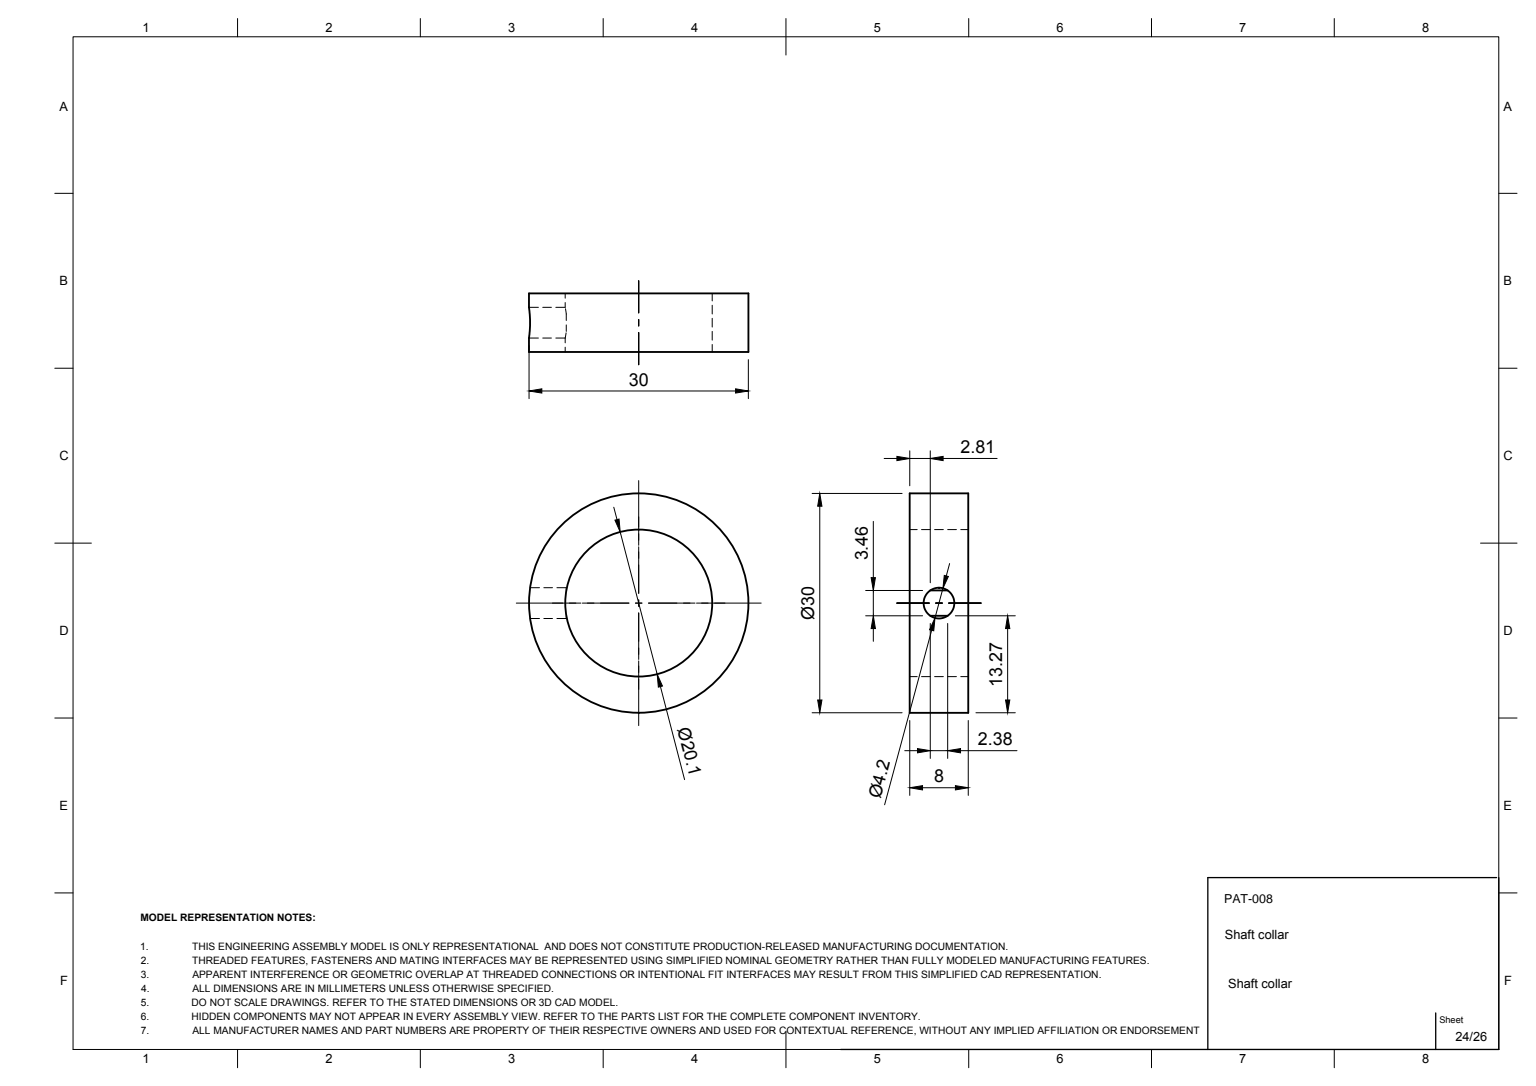
ISO-10303-21;
HEADER;
/* Generated by software containing ST-Developer
 * from STEP Tools, Inc. (www.steptools.com) 
 */

FILE_DESCRIPTION(
/* description */ ('Bearing housing with oil seal and end cap'),
/* implementation_level */ '2;1');

FILE_NAME(
/* name */ 'Shaft collar.step',
/* time_stamp */ '2026-10-28T03:23:10-07:00',
/* author */ (''),
/* organization */ (''),
/* preprocessor_version */ 'ST-DEVELOPER v20.2',
/* originating_system */ 'Autodesk Translation Framework v15.17.0.0',
/* authorisation */ '');

FILE_SCHEMA (('AUTOMOTIVE_DESIGN { 1 0 10303 214 3 1 1 }'));
ENDSEC;

DATA;
#10=MECHANICAL_DESIGN_GEOMETRIC_PRESENTATION_REPRESENTATION('',(#284),#7871);
#177=B_SPLINE_CURVE_WITH_KNOTS('',3,(#7483,#7484,#7485,#7486,#7487,#7488,
#7489,#7490,#7491,#7492,#7493,#7494,#7495,#7496),.UNSPECIFIED.,.F.,.F.,
(4,2,2,2,2,2,4),(0.756005737987012,0.793568827564648,0.872922520054202,
0.952276212543757,1.03162990503331,1.11098359752287,1.1485466871005),
 .UNSPECIFIED.);
#178=B_SPLINE_CURVE_WITH_KNOTS('',3,(#7502,#7503,#7504,#7505,#7506,#7507,
#7508,#7509,#7510,#7511,#7512,#7513,#7514,#7515,#7516,#7517,#7518,#7519),
 .UNSPECIFIED.,.F.,.F.,(4,2,2,2,2,2,2,2,4),(0.,0.0792165807733632,0.158433161546726,
0.237648697074571,0.316864232602415,0.396079768130259,0.475295303658103,
0.554511884431466,0.63372846520483),.UNSPECIFIED.);
#179=B_SPLINE_CURVE_WITH_KNOTS('',3,(#7520,#7521,#7522,#7523,#7524,#7525,
#7526,#7527,#7528,#7529,#7530,#7531,#7532,#7533,#7534,#7535,#7536,#7537),
 .UNSPECIFIED.,.F.,.F.,(4,2,2,2,2,2,2,2,4),(0.63372846520483,0.712945045978192,
0.792161626751555,0.8713771622794,0.950592697807244,1.02980823333509,1.10902376886293,
1.1882403496363,1.26745693040966),.UNSPECIFIED.);
#180=B_SPLINE_CURVE_WITH_KNOTS('',3,(#7540,#7541,#7542,#7543,#7544,#7545,
#7546,#7547,#7548,#7549,#7550,#7551,#7552,#7553),.UNSPECIFIED.,.F.,.F.,
(4,2,2,2,2,2,4),(0.121154929624506,0.158718019202143,0.238071711691698,
0.317425404181252,0.396779096670807,0.476132789160362,0.513695878737999),
 .UNSPECIFIED.);
#234=SHAPE_REPRESENTATION_RELATIONSHIP('SRR','None',#7983,#255);
#255=ADVANCED_BREP_SHAPE_REPRESENTATION('',(#311),#7867);
#284=STYLED_ITEM('',(#8153),#311);
#311=MANIFOLD_SOLID_BREP('Body1',#4112);
#390=FACE_BOUND('',#1088,.T.);
#391=FACE_BOUND('',#1090,.T.);
#392=FACE_BOUND('',#1092,.T.);
#393=FACE_BOUND('',#1094,.T.);
#521=PLANE('',#4795);
#522=PLANE('',#4800);
#523=PLANE('',#4807);
#524=PLANE('',#4808);
#758=FACE_OUTER_BOUND('',#1084,.T.);
#759=FACE_OUTER_BOUND('',#1085,.T.);
#760=FACE_OUTER_BOUND('',#1086,.T.);
#761=FACE_OUTER_BOUND('',#1087,.T.);
#762=FACE_OUTER_BOUND('',#1089,.T.);
#763=FACE_OUTER_BOUND('',#1091,.T.);
#764=FACE_OUTER_BOUND('',#1093,.T.);
#1084=EDGE_LOOP('',(#3549,#3550));
#1085=EDGE_LOOP('',(#3551,#3552,#3553,#3554,#3555,#3556,#3557,#3558,#3559));
#1086=EDGE_LOOP('',(#3560,#3561,#3562));
#1087=EDGE_LOOP('',(#3563,#3564,#3565,#3566));
#1088=EDGE_LOOP('',(#3567,#3568,#3569,#3570));
#1089=EDGE_LOOP('',(#3571,#3572,#3573,#3574));
#1090=EDGE_LOOP('',(#3575,#3576));
#1091=EDGE_LOOP('',(#3577));
#1092=EDGE_LOOP('',(#3578));
#1093=EDGE_LOOP('',(#3579));
#1094=EDGE_LOOP('',(#3580));
#1340=LINE('',#7479,#1602);
#1341=LINE('',#7500,#1603);
#1342=LINE('',#7555,#1604);
#1343=LINE('',#7560,#1605);
#1344=LINE('',#7566,#1606);
#1602=VECTOR('',#5969,1.);
#1603=VECTOR('',#5976,0.21);
#1604=VECTOR('',#5981,1.);
#1605=VECTOR('',#5986,1.005);
#1606=VECTOR('',#5993,1.5);
#1863=CIRCLE('',#4796,0.21);
#1864=CIRCLE('',#4798,0.21);
#1865=CIRCLE('',#4799,0.21);
#1866=CIRCLE('',#4802,1.005);
#1867=CIRCLE('',#4803,1.005);
#1868=CIRCLE('',#4805,1.5);
#1869=CIRCLE('',#4806,1.5);
#2165=VERTEX_POINT('',#7477);
#2166=VERTEX_POINT('',#7478);
#2167=VERTEX_POINT('',#7482);
#2168=VERTEX_POINT('',#7497);
#2169=VERTEX_POINT('',#7499);
#2170=VERTEX_POINT('',#7501);
#2171=VERTEX_POINT('',#7538);
#2172=VERTEX_POINT('',#7557);
#2173=VERTEX_POINT('',#7559);
#2174=VERTEX_POINT('',#7563);
#2175=VERTEX_POINT('',#7565);
#2638=EDGE_CURVE('',#2165,#2166,#1340,.T.);
#2639=EDGE_CURVE('',#2165,#2166,#1863,.T.);
#2640=EDGE_CURVE('',#2167,#2165,#177,.T.);
#2641=EDGE_CURVE('',#2168,#2167,#1864,.T.);
#2642=EDGE_CURVE('',#2168,#2169,#1341,.T.);
#2643=EDGE_CURVE('',#2170,#2169,#178,.T.);
#2644=EDGE_CURVE('',#2169,#2170,#179,.T.);
#2645=EDGE_CURVE('',#2171,#2168,#1865,.T.);
#2646=EDGE_CURVE('',#2166,#2171,#180,.T.);
#2647=EDGE_CURVE('',#2171,#2167,#1342,.T.);
#2648=EDGE_CURVE('',#2172,#2172,#1866,.T.);
#2649=EDGE_CURVE('',#2172,#2173,#1343,.T.);
#2650=EDGE_CURVE('',#2173,#2173,#1867,.T.);
#2651=EDGE_CURVE('',#2174,#2174,#1868,.T.);
#2652=EDGE_CURVE('',#2174,#2175,#1344,.T.);
#2653=EDGE_CURVE('',#2175,#2175,#1869,.T.);
#3549=ORIENTED_EDGE('',*,*,#2638,.F.);
#3550=ORIENTED_EDGE('',*,*,#2639,.T.);
#3551=ORIENTED_EDGE('',*,*,#2640,.F.);
#3552=ORIENTED_EDGE('',*,*,#2641,.F.);
#3553=ORIENTED_EDGE('',*,*,#2642,.T.);
#3554=ORIENTED_EDGE('',*,*,#2643,.F.);
#3555=ORIENTED_EDGE('',*,*,#2644,.F.);
#3556=ORIENTED_EDGE('',*,*,#2642,.F.);
#3557=ORIENTED_EDGE('',*,*,#2645,.F.);
#3558=ORIENTED_EDGE('',*,*,#2646,.F.);
#3559=ORIENTED_EDGE('',*,*,#2639,.F.);
#3560=ORIENTED_EDGE('',*,*,#2647,.F.);
#3561=ORIENTED_EDGE('',*,*,#2645,.T.);
#3562=ORIENTED_EDGE('',*,*,#2641,.T.);
#3563=ORIENTED_EDGE('',*,*,#2648,.F.);
#3564=ORIENTED_EDGE('',*,*,#2649,.T.);
#3565=ORIENTED_EDGE('',*,*,#2650,.T.);
#3566=ORIENTED_EDGE('',*,*,#2649,.F.);
#3567=ORIENTED_EDGE('',*,*,#2646,.T.);
#3568=ORIENTED_EDGE('',*,*,#2647,.T.);
#3569=ORIENTED_EDGE('',*,*,#2640,.T.);
#3570=ORIENTED_EDGE('',*,*,#2638,.T.);
#3571=ORIENTED_EDGE('',*,*,#2651,.F.);
#3572=ORIENTED_EDGE('',*,*,#2652,.T.);
#3573=ORIENTED_EDGE('',*,*,#2653,.T.);
#3574=ORIENTED_EDGE('',*,*,#2652,.F.);
#3575=ORIENTED_EDGE('',*,*,#2643,.T.);
#3576=ORIENTED_EDGE('',*,*,#2644,.T.);
#3577=ORIENTED_EDGE('',*,*,#2651,.T.);
#3578=ORIENTED_EDGE('',*,*,#2648,.T.);
#3579=ORIENTED_EDGE('',*,*,#2653,.F.);
#3580=ORIENTED_EDGE('',*,*,#2650,.F.);
#3822=CYLINDRICAL_SURFACE('',#4797,0.21);
#3823=CYLINDRICAL_SURFACE('',#4801,1.005);
#3824=CYLINDRICAL_SURFACE('',#4804,1.5);
#4040=ADVANCED_FACE('',(#758),#521,.T.);
#4041=ADVANCED_FACE('',(#759),#3822,.F.);
#4042=ADVANCED_FACE('',(#760),#522,.T.);
#4043=ADVANCED_FACE('',(#761,#390),#3823,.F.);
#4044=ADVANCED_FACE('',(#762,#391),#3824,.T.);
#4045=ADVANCED_FACE('',(#763,#392),#523,.T.);
#4046=ADVANCED_FACE('',(#764,#393),#524,.F.);
#4112=CLOSED_SHELL('',(#4040,#4041,#4042,#4043,#4044,#4045,#4046));
#4794=AXIS2_PLACEMENT_3D('',#7475,#5965,#5966);
#4795=AXIS2_PLACEMENT_3D('',#7476,#5967,#5968);
#4796=AXIS2_PLACEMENT_3D('',#7480,#5970,#5971);
#4797=AXIS2_PLACEMENT_3D('',#7481,#5972,#5973);
#4798=AXIS2_PLACEMENT_3D('',#7498,#5974,#5975);
#4799=AXIS2_PLACEMENT_3D('',#7539,#5977,#5978);
#4800=AXIS2_PLACEMENT_3D('',#7554,#5979,#5980);
#4801=AXIS2_PLACEMENT_3D('',#7556,#5982,#5983);
#4802=AXIS2_PLACEMENT_3D('',#7558,#5984,#5985);
#4803=AXIS2_PLACEMENT_3D('',#7561,#5987,#5988);
#4804=AXIS2_PLACEMENT_3D('',#7562,#5989,#5990);
#4805=AXIS2_PLACEMENT_3D('',#7564,#5991,#5992);
#4806=AXIS2_PLACEMENT_3D('',#7567,#5994,#5995);
#4807=AXIS2_PLACEMENT_3D('',#7568,#5996,#5997);
#4808=AXIS2_PLACEMENT_3D('',#7569,#5998,#5999);
#5965=DIRECTION('axis',(0.,0.,1.));
#5966=DIRECTION('refdir',(1.,0.,0.));
#5967=DIRECTION('center_axis',(0.,0.,1.));
#5968=DIRECTION('ref_axis',(1.,0.,0.));
#5969=DIRECTION('',(0.,1.,0.));
#5970=DIRECTION('center_axis',(0.,0.,1.));
#5971=DIRECTION('ref_axis',(1.,0.,0.));
#5972=DIRECTION('center_axis',(0.,0.,1.));
#5973=DIRECTION('ref_axis',(1.,0.,0.));
#5974=DIRECTION('center_axis',(0.,0.,1.));
#5975=DIRECTION('ref_axis',(1.,0.,0.));
#5976=DIRECTION('',(0.,0.,1.));
#5977=DIRECTION('center_axis',(0.,0.,1.));
#5978=DIRECTION('ref_axis',(1.,0.,0.));
#5979=DIRECTION('center_axis',(0.,0.,1.));
#5980=DIRECTION('ref_axis',(1.,0.,0.));
#5981=DIRECTION('',(0.,-1.,0.));
#5982=DIRECTION('center_axis',(0.,1.,0.));
#5983=DIRECTION('ref_axis',(1.,0.,0.));
#5984=DIRECTION('center_axis',(0.,-1.,0.));
#5985=DIRECTION('ref_axis',(1.,0.,0.));
#5986=DIRECTION('',(0.,-1.,0.));
#5987=DIRECTION('center_axis',(0.,-1.,0.));
#5988=DIRECTION('ref_axis',(1.,0.,0.));
#5989=DIRECTION('center_axis',(0.,1.,0.));
#5990=DIRECTION('ref_axis',(1.,0.,0.));
#5991=DIRECTION('center_axis',(0.,1.,0.));
#5992=DIRECTION('ref_axis',(1.,0.,0.));
#5993=DIRECTION('',(0.,-1.,0.));
#5994=DIRECTION('center_axis',(0.,1.,0.));
#5995=DIRECTION('ref_axis',(1.,0.,0.));
#5996=DIRECTION('center_axis',(0.,1.,0.));
#5997=DIRECTION('ref_axis',(1.,0.,0.));
#5998=DIRECTION('center_axis',(0.,1.,0.));
#5999=DIRECTION('ref_axis',(1.,0.,0.));
#7475=CARTESIAN_POINT('',(0.,0.,0.));
#7476=CARTESIAN_POINT('Origin',(0.,6.4,5.49));
#7477=CARTESIAN_POINT('',(0.172988438920061,6.28094119100209,5.49));
#7478=CARTESIAN_POINT('',(0.172988438920061,6.51905880899791,5.49));
#7479=CARTESIAN_POINT('',(0.172988438920061,6.,5.49));
#7480=CARTESIAN_POINT('Origin',(0.,6.4,5.49));
#7481=CARTESIAN_POINT('Origin',(0.,6.4,5.49));
#7482=CARTESIAN_POINT('',(-0.172988438920061,6.28094119100209,5.49));
#7483=CARTESIAN_POINT('Ctrl Pts',(-0.172988438920061,6.28094119100209,5.49));
#7484=CARTESIAN_POINT('Ctrl Pts',(-0.165594865311318,6.27019857760471,5.49129192197638));
#7485=CARTESIAN_POINT('Ctrl Pts',(-0.157297138725608,6.26031229062726,5.49265394943905));
#7486=CARTESIAN_POINT('Ctrl Pts',(-0.129892073845076,6.23290722574673,5.4967480843909));
#7487=CARTESIAN_POINT('Ctrl Pts',(-0.106330167759284,6.21675794366705,5.49969589327638));
#7488=CARTESIAN_POINT('Ctrl Pts',(-0.05461290463241,6.19530220603509,5.50385029472357));
#7489=CARTESIAN_POINT('Ctrl Pts',(-0.0264512308298516,6.19,5.505));
#7490=CARTESIAN_POINT('Ctrl Pts',(0.0264512308298515,6.19,5.505));
#7491=CARTESIAN_POINT('Ctrl Pts',(0.0546129046324099,6.19530220603509,5.50385029472357));
#7492=CARTESIAN_POINT('Ctrl Pts',(0.106330167759284,6.21675794366705,5.49969589327638));
#7493=CARTESIAN_POINT('Ctrl Pts',(0.129892073845076,6.23290722574673,5.4967480843909));
#7494=CARTESIAN_POINT('Ctrl Pts',(0.157297138725608,6.26031229062726,5.49265394943905));
#7495=CARTESIAN_POINT('Ctrl Pts',(0.165594865311318,6.27019857760471,5.49129192197638));
#7496=CARTESIAN_POINT('Ctrl Pts',(0.172988438920061,6.28094119100209,5.49));
#7497=CARTESIAN_POINT('',(-0.21,6.4,5.49));
#7498=CARTESIAN_POINT('Origin',(0.,6.4,5.49));
#7499=CARTESIAN_POINT('',(-0.21,6.4,5.98522725533839));
#7500=CARTESIAN_POINT('',(-0.21,6.4,5.49));
#7501=CARTESIAN_POINT('',(0.21,6.4,5.98522725533839));
#7502=CARTESIAN_POINT('Ctrl Pts',(0.21,6.4,5.98522725533839));
#7503=CARTESIAN_POINT('Ctrl Pts',(0.21,6.37359447307555,5.98522725533839));
#7504=CARTESIAN_POINT('Ctrl Pts',(0.204715737269596,6.34545292590929,5.98600415954412));
#7505=CARTESIAN_POINT('Ctrl Pts',(0.183273763036332,6.29372373109487,5.98880073282317));
#7506=CARTESIAN_POINT('Ctrl Pts',(0.167117923970394,6.27013307587204,5.99077897157582));
#7507=CARTESIAN_POINT('Ctrl Pts',(0.129867169887369,6.23288232178902,5.99448481141327));
#7508=CARTESIAN_POINT('Ctrl Pts',(0.106276408305765,6.21672628999865,5.99645455657129));
#7509=CARTESIAN_POINT('Ctrl Pts',(0.0545468514059002,6.19528417517378,5.99923165515646));
#7510=CARTESIAN_POINT('Ctrl Pts',(0.0264051785092814,6.19,6.));
#7511=CARTESIAN_POINT('Ctrl Pts',(-0.0264051785092814,6.19,6.));
#7512=CARTESIAN_POINT('Ctrl Pts',(-0.0545468514059002,6.19528417517378,
5.99923165515646));
#7513=CARTESIAN_POINT('Ctrl Pts',(-0.106276408305765,6.21672628999865,5.99645455657129));
#7514=CARTESIAN_POINT('Ctrl Pts',(-0.129867169887369,6.23288232178902,5.99448481141327));
#7515=CARTESIAN_POINT('Ctrl Pts',(-0.167117923970394,6.27013307587204,5.99077897157582));
#7516=CARTESIAN_POINT('Ctrl Pts',(-0.183273763036332,6.29372373109487,5.98880073282317));
#7517=CARTESIAN_POINT('Ctrl Pts',(-0.204715737269596,6.34545292590929,5.98600415954412));
#7518=CARTESIAN_POINT('Ctrl Pts',(-0.21,6.37359447307555,5.98522725533839));
#7519=CARTESIAN_POINT('Ctrl Pts',(-0.21,6.4,5.98522725533839));
#7520=CARTESIAN_POINT('Ctrl Pts',(-0.21,6.4,5.98522725533839));
#7521=CARTESIAN_POINT('Ctrl Pts',(-0.21,6.42640552692446,5.98522725533839));
#7522=CARTESIAN_POINT('Ctrl Pts',(-0.204715737269596,6.45454707409071,5.98600415954412));
#7523=CARTESIAN_POINT('Ctrl Pts',(-0.183273763036332,6.50627626890513,5.98880073282317));
#7524=CARTESIAN_POINT('Ctrl Pts',(-0.167117923970394,6.52986692412796,5.99077897157582));
#7525=CARTESIAN_POINT('Ctrl Pts',(-0.129867169887369,6.56711767821098,5.99448481141327));
#7526=CARTESIAN_POINT('Ctrl Pts',(-0.106276408305765,6.58327371000135,5.99645455657129));
#7527=CARTESIAN_POINT('Ctrl Pts',(-0.0545468514059003,6.60471582482622,
5.99923165515646));
#7528=CARTESIAN_POINT('Ctrl Pts',(-0.0264051785092815,6.61,6.));
#7529=CARTESIAN_POINT('Ctrl Pts',(0.0264051785092814,6.61,6.));
#7530=CARTESIAN_POINT('Ctrl Pts',(0.0545468514059006,6.60471582482622,5.99923165515646));
#7531=CARTESIAN_POINT('Ctrl Pts',(0.106276408305766,6.58327371000135,5.99645455657129));
#7532=CARTESIAN_POINT('Ctrl Pts',(0.129867169887369,6.56711767821098,5.99448481141327));
#7533=CARTESIAN_POINT('Ctrl Pts',(0.167117923970393,6.52986692412796,5.99077897157582));
#7534=CARTESIAN_POINT('Ctrl Pts',(0.183273763036332,6.50627626890513,5.98880073282317));
#7535=CARTESIAN_POINT('Ctrl Pts',(0.204715737269596,6.45454707409071,5.98600415954412));
#7536=CARTESIAN_POINT('Ctrl Pts',(0.21,6.42640552692446,5.98522725533839));
#7537=CARTESIAN_POINT('Ctrl Pts',(0.21,6.4,5.98522725533839));
#7538=CARTESIAN_POINT('',(-0.172988438920061,6.51905880899791,5.49));
#7539=CARTESIAN_POINT('Origin',(0.,6.4,5.49));
#7540=CARTESIAN_POINT('Ctrl Pts',(0.172988438920061,6.51905880899791,5.49));
#7541=CARTESIAN_POINT('Ctrl Pts',(0.165594865311319,6.52980142239529,5.49129192197638));
#7542=CARTESIAN_POINT('Ctrl Pts',(0.157297138725609,6.53968770937274,5.49265394943905));
#7543=CARTESIAN_POINT('Ctrl Pts',(0.129892073845076,6.56709277425327,5.4967480843909));
#7544=CARTESIAN_POINT('Ctrl Pts',(0.106330167759284,6.58324205633295,5.49969589327638));
#7545=CARTESIAN_POINT('Ctrl Pts',(0.05461290463241,6.60469779396491,5.50385029472357));
#7546=CARTESIAN_POINT('Ctrl Pts',(0.0264512308298516,6.61,5.505));
#7547=CARTESIAN_POINT('Ctrl Pts',(-0.0264512308298515,6.61,5.505));
#7548=CARTESIAN_POINT('Ctrl Pts',(-0.05461290463241,6.60469779396491,5.50385029472357));
#7549=CARTESIAN_POINT('Ctrl Pts',(-0.106330167759284,6.58324205633295,5.49969589327638));
#7550=CARTESIAN_POINT('Ctrl Pts',(-0.129892073845076,6.56709277425328,5.4967480843909));
#7551=CARTESIAN_POINT('Ctrl Pts',(-0.157297138725609,6.53968770937274,5.49265394943905));
#7552=CARTESIAN_POINT('Ctrl Pts',(-0.165594865311318,6.52980142239529,5.49129192197638));
#7553=CARTESIAN_POINT('Ctrl Pts',(-0.172988438920062,6.51905880899791,5.49));
#7554=CARTESIAN_POINT('Origin',(0.,6.4,5.49));
#7555=CARTESIAN_POINT('',(-0.172988438920061,6.,5.49));
#7556=CARTESIAN_POINT('Origin',(0.,6.,4.5));
#7557=CARTESIAN_POINT('',(-1.005,6.8,4.5));
#7558=CARTESIAN_POINT('Origin',(0.,6.8,4.5));
#7559=CARTESIAN_POINT('',(-1.005,6.,4.5));
#7560=CARTESIAN_POINT('',(-1.005,6.,4.5));
#7561=CARTESIAN_POINT('Origin',(0.,6.,4.5));
#7562=CARTESIAN_POINT('Origin',(0.,6.,4.5));
#7563=CARTESIAN_POINT('',(-1.5,6.8,4.5));
#7564=CARTESIAN_POINT('Origin',(0.,6.8,4.5));
#7565=CARTESIAN_POINT('',(-1.5,6.,4.5));
#7566=CARTESIAN_POINT('',(-1.5,6.,4.5));
#7567=CARTESIAN_POINT('Origin',(0.,6.,4.5));
#7568=CARTESIAN_POINT('Origin',(0.,6.8,4.5));
#7569=CARTESIAN_POINT('Origin',(0.,6.,4.5));
#7841=UNCERTAINTY_MEASURE_WITH_UNIT(LENGTH_MEASURE(0.001),#7872,
'DISTANCE_ACCURACY_VALUE',
'Maximum model space distance between geometric entities at asserted c
onnectivities');
#7845=UNCERTAINTY_MEASURE_WITH_UNIT(LENGTH_MEASURE(0.001),#7872,
'DISTANCE_ACCURACY_VALUE',
'Maximum model space distance between geometric entities at asserted c
onnectivities');
#7867=(
GEOMETRIC_REPRESENTATION_CONTEXT(3)
GLOBAL_UNCERTAINTY_ASSIGNED_CONTEXT((#7841))
GLOBAL_UNIT_ASSIGNED_CONTEXT((#7872,#7874,#7875))
REPRESENTATION_CONTEXT('','3D')
);
#7871=(
GEOMETRIC_REPRESENTATION_CONTEXT(3)
GLOBAL_UNCERTAINTY_ASSIGNED_CONTEXT((#7845))
GLOBAL_UNIT_ASSIGNED_CONTEXT((#7872,#7874,#7875))
REPRESENTATION_CONTEXT('','3D')
);
#7872=(
LENGTH_UNIT()
NAMED_UNIT(*)
SI_UNIT(.CENTI.,.METRE.)
);
#7874=(
NAMED_UNIT(*)
PLANE_ANGLE_UNIT()
SI_UNIT($,.RADIAN.)
);
#7875=(
NAMED_UNIT(*)
SI_UNIT($,.STERADIAN.)
SOLID_ANGLE_UNIT()
);
#7897=SHAPE_DEFINITION_REPRESENTATION(#7949,#7983);
#7949=PRODUCT_DEFINITION_SHAPE('',$,#8009);
#7983=SHAPE_REPRESENTATION('',(#4794),#7867);
#7987=PRODUCT_DEFINITION_CONTEXT('part definition',#8064,'design');
#8009=PRODUCT_DEFINITION('Shaft collar','Shaft collar',#8034,#7987);
#8034=PRODUCT_DEFINITION_FORMATION('',$,#8087);
#8064=APPLICATION_CONTEXT(
'Core Data for Automotive Mechanical Design Process');
#8065=PRODUCT_CONTEXT('part definition',#8064,'mechanical');
#8087=PRODUCT('Shaft collar','Shaft collar','Shaft collar',(#8065));
#8147=COLOUR_RGB('Grey',0.48,0.52,0.57);
#8148=FILL_AREA_STYLE_COLOUR('',#8147);
#8149=FILL_AREA_STYLE('',(#8148));
#8150=SURFACE_STYLE_FILL_AREA(#8149);
#8151=SURFACE_SIDE_STYLE('',(#8150));
#8152=SURFACE_STYLE_USAGE(.BOTH.,#8151);
#8153=PRESENTATION_STYLE_ASSIGNMENT((#8152));
ENDSEC;
END-ISO-10303-21;
